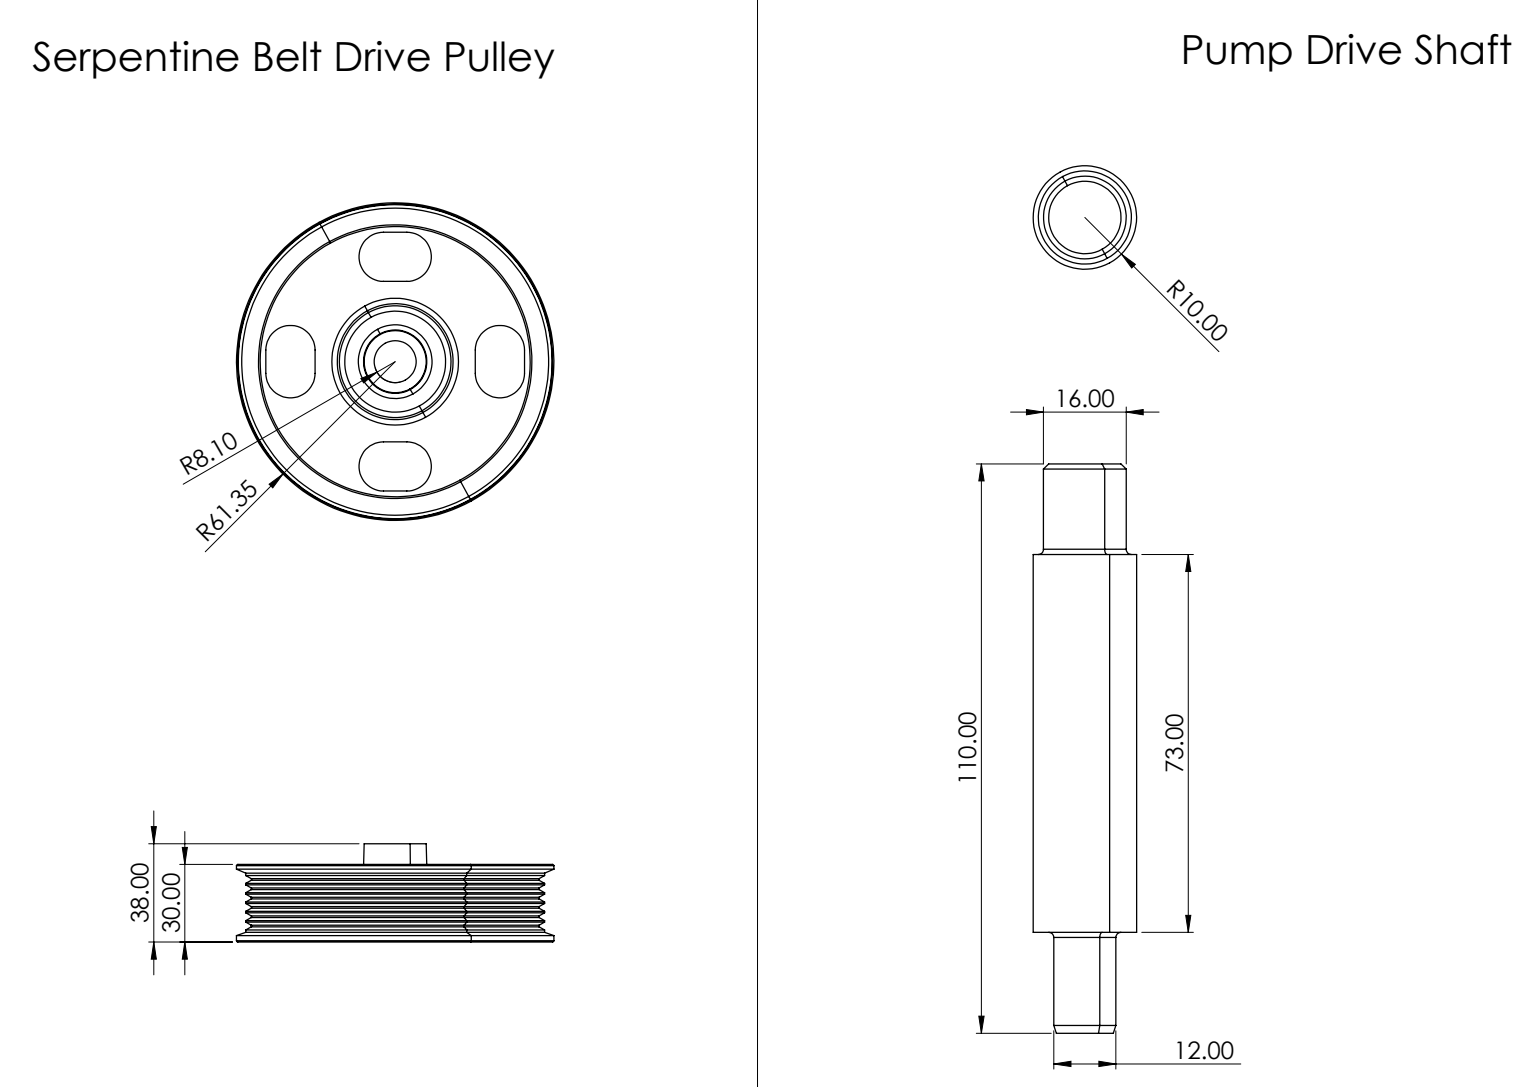
ISO-10303-21;
HEADER;
FILE_DESCRIPTION (('STEP AP214'),
    '1' );
FILE_NAME ('Pump Drive Shaft.step',
    '2026-10-09T13:19:41',
    ( '' ),
    ( '' ),
    'SwSTEP 2.0',
    'SolidWorks 2026',
    '' );
FILE_SCHEMA (( 'AUTOMOTIVE_DESIGN' ));
ENDSEC;

DATA;
#39=AXIS2_PLACEMENT_3D ( 'NONE', #26145, #6457, #10384 ) ;
#47=EDGE_CURVE ( 'NONE', #418, #1224, #23072, .T. ) ;
#183=CARTESIAN_POINT ( 'NONE',  ( 0.000000000000000000, 4.440892098500000496E-16, 0.000000000000000000 ) ) ;
#309=EDGE_LOOP ( 'NONE', ( #11613, #26788, #16517, #882 ) ) ;
#314=DIRECTION ( 'NONE',  ( 0.000000000000000000, -1.000000000000000000, 0.000000000000000000 ) ) ;
#372=DIRECTION ( 'NONE',  ( 0.000000000000000000, 1.000000000000000000, 0.000000000000000000 ) ) ;
#400=VERTEX_POINT ( 'NONE', #13649 ) ;
#418=VERTEX_POINT ( 'NONE', #2300 ) ;
#420=CARTESIAN_POINT ( 'NONE',  ( 0.000000000000000000, -90.50000000000000000, 0.000000000000000000 ) ) ;
#477=CYLINDRICAL_SURFACE ( 'NONE', #16417, 5.999999999999999112 ) ;
#489=LINE ( 'NONE', #22764, #1160 ) ;
#536=CONICAL_SURFACE ( 'NONE', #26096, 7.000000000000005329, 0.7853981633970000820 ) ;
#605=ADVANCED_FACE ( 'NONE', ( #18903 ), #27359, .T. ) ;
#882=ORIENTED_EDGE ( 'NONE', *, *, #11910, .F. ) ;
#893=CARTESIAN_POINT ( 'NONE',  ( -4.314829847440000421, -16.50000000000000000, -7.898243057010000179 ) ) ;
#942=VECTOR ( 'NONE', #24106, 999.9999999999998863 ) ;
#989=ORIENTED_EDGE ( 'NONE', *, *, #21743, .T. ) ;
#1012=CYLINDRICAL_SURFACE ( 'NONE', #26910, 9.999999999999996447 ) ;
#1058=DIRECTION ( 'NONE',  ( 0.000000000000000000, 1.000000000000000000, 0.000000000000000000 ) ) ;
#1160=VECTOR ( 'NONE', #22914, 1000.000000000000000 ) ;
#1187=VERTEX_POINT ( 'NONE', #12940 ) ;
#1224=VERTEX_POINT ( 'NONE', #14279 ) ;
#1275=DIRECTION ( 'NONE',  ( 1.000000000000000000, 0.000000000000000000, 0.000000000000000000 ) ) ;
#1309=PRODUCT ( 'Pump Drive Shaft', 'Pump Drive Shaft', '', ( #7289 ) ) ;
#1335=CARTESIAN_POINT ( 'NONE',  ( 0.000000000000000000, -90.50000000000000000, 0.000000000000000000 ) ) ;
#1353=DIRECTION ( 'NONE',  ( 0.4794255386042041156, 0.000000000000000000, 0.8775825618903722036 ) ) ;
#1356=LINE ( 'NONE', #11841, #17621 ) ;
#1363=ORIENTED_EDGE ( 'NONE', *, *, #7055, .F. ) ;
#1508=ORIENTED_EDGE ( 'NONE', *, *, #11910, .T. ) ;
#1532=ORIENTED_EDGE ( 'NONE', *, *, #17302, .F. ) ;
#1603=CONICAL_SURFACE ( 'NONE', #17400, 5.499999999999999112, 0.3217505543970000104 ) ;
#1714=FACE_OUTER_BOUND ( 'NONE', #309, .T. ) ;
#1771=DIRECTION ( 'NONE',  ( 0.000000000000000000, 1.000000000000000000, 0.000000000000000000 ) ) ;
#1915=DIRECTION ( 'NONE',  ( 0.000000000000000000, 1.000000000000000000, 0.000000000000000000 ) ) ;
#2006=SURFACE_STYLE_USAGE ( .BOTH. , #21957 ) ;
#2018=SHAPE_REPRESENTATION ( 'Pump Drive Shaft', ( #26433 ), #4100 ) ;
#2091=ADVANCED_FACE ( 'NONE', ( #11496 ), #477, .T. ) ;
#2175=CARTESIAN_POINT ( 'NONE',  ( 0.000000000000000000, -17.50000000000000000, 9.000000000000000000 ) ) ;
#2277=ADVANCED_FACE ( 'NONE', ( #17754 ), #24157, .F. ) ;
#2300=CARTESIAN_POINT ( 'NONE',  ( -2.636840462319999912, -110.0000000000000000, -4.826704090399999814 ) ) ;
#2315=ORIENTED_EDGE ( 'NONE', *, *, #7596, .T. ) ;
#2374=DIRECTION ( 'NONE',  ( 0.000000000000000000, 1.000000000000000000, 0.000000000000000000 ) ) ;
#2485=LINE ( 'NONE', #11341, #28396 ) ;
#2669=( NAMED_UNIT ( * ) PLANE_ANGLE_UNIT ( ) SI_UNIT ( $, .RADIAN. ) );
#2893=CONICAL_SURFACE ( 'NONE', #7090, 5.499999999999999112, 0.3217505543970000104 ) ;
#2930=CARTESIAN_POINT ( 'NONE',  ( -3.595691539529999758, -0.5000000000000000000, -6.581869214180000149 ) ) ;
#2950=DIRECTION ( 'NONE',  ( 0.000000000000000000, 1.000000000000000000, 0.000000000000000000 ) ) ;
#3005=AXIS2_PLACEMENT_3D ( 'NONE', #25732, #25170, #16694 ) ;
#3020=ORIENTED_EDGE ( 'NONE', *, *, #21743, .F. ) ;
#3033=EDGE_LOOP ( 'NONE', ( #27867, #12027, #6228, #27507 ) ) ;
#3034=AXIS2_PLACEMENT_3D ( 'NONE', #12319, #16700, #27659 ) ;
#3057=CARTESIAN_POINT ( 'NONE',  ( 0.000000000000000000, -90.50000000000000000, 0.000000000000000000 ) ) ;
#3314=AXIS2_PLACEMENT_3D ( 'NONE', #893, #16880, #19198 ) ;
#3446=CIRCLE ( 'NONE', #15027, 6.000000000000000000 ) ;
#3603=DIRECTION ( 'NONE',  ( 0.4794255386042040601, 0.000000000000000000, 0.8775825618903720926 ) ) ;
#3619=PRODUCT_DEFINITION_CONTEXT ( 'detailed design', #11839, 'design' ) ;
#3643=DIRECTION ( 'NONE',  ( 0.000000000000000000, 1.000000000000000000, 0.000000000000000000 ) ) ;
#3653=PRODUCT_DEFINITION_FORMATION_WITH_SPECIFIED_SOURCE ( 'ANY', '', #1309, .NOT_KNOWN. ) ;
#3670=ORIENTED_EDGE ( 'NONE', *, *, #26322, .F. ) ;
#3706=DIRECTION ( 'NONE',  ( 0.000000000000000000, 1.000000000000000000, 0.000000000000000000 ) ) ;
#3751=CARTESIAN_POINT ( 'NONE',  ( 0.000000000000000000, -110.0000000000000000, 0.000000000000000000 ) ) ;
#3889=DIRECTION ( 'NONE',  ( 1.000000000000000000, 0.000000000000000000, 0.000000000000000000 ) ) ;
#4040=ORIENTED_EDGE ( 'NONE', *, *, #20407, .T. ) ;
#4065=ADVANCED_FACE ( 'NONE', ( #10873, #19783 ), #17613, .T. ) ;
#4100=( GEOMETRIC_REPRESENTATION_CONTEXT ( 3 ) GLOBAL_UNCERTAINTY_ASSIGNED_CONTEXT ( ( #25217 ) ) GLOBAL_UNIT_ASSIGNED_CONTEXT ( ( #7186, #2669, #27289 ) ) REPRESENTATION_CONTEXT ( 'NONE', 'WORKASPACE' ) );
#4149=DIRECTION ( 'NONE',  ( 1.000000000000000000, 0.000000000000000000, 0.000000000000000000 ) ) ;
#4189=AXIS2_PLACEMENT_3D ( 'NONE', #19021, #12432, #23257 ) ;
#4211=DIRECTION ( 'NONE',  ( 0.000000000000000000, 1.000000000000000000, 0.000000000000000000 ) ) ;
#4213=TOROIDAL_SURFACE ( 'NONE', #5625, 9.000000000000000000, 1.000000000000000000 ) ;
#4271=VERTEX_POINT ( 'NONE', #17004 ) ;
#4384=DIRECTION ( 'NONE',  ( 0.000000000000000000, 1.000000000000000000, 0.000000000000000000 ) ) ;
#4492=DIRECTION ( 'NONE',  ( 0.4794255386042036715, 0.000000000000000000, 0.8775825618903724257 ) ) ;
#4610=ORIENTED_EDGE ( 'NONE', *, *, #24145, .F. ) ;
#4642=FACE_OUTER_BOUND ( 'NONE', #3033, .T. ) ;
#4769=VERTEX_POINT ( 'NONE', #9862 ) ;
#4778=ORIENTED_EDGE ( 'NONE', *, *, #20355, .F. ) ;
#4784=VERTEX_POINT ( 'NONE', #6974 ) ;
#4813=AXIS2_PLACEMENT_3D ( 'NONE', #183, #4384, #22460 ) ;
#4816=EDGE_LOOP ( 'NONE', ( #20575, #7039 ) ) ;
#4866=DIRECTION ( 'NONE',  ( 0.4794255386042041156, 0.000000000000000000, 0.8775825618903722036 ) ) ;
#5178=DIRECTION ( 'NONE',  ( 1.000000000000000000, 0.000000000000000000, 0.000000000000000000 ) ) ;
#5246=ORIENTED_EDGE ( 'NONE', *, *, #8164, .T. ) ;
#5297=FACE_OUTER_BOUND ( 'NONE', #22057, .T. ) ;
#5300=AXIS2_PLACEMENT_3D ( 'NONE', #17761, #26647, #4492 ) ;
#5306=ORIENTED_EDGE ( 'NONE', *, *, #15873, .T. ) ;
#5347=DIRECTION ( 'NONE',  ( 1.000000000000000000, 0.000000000000000000, 0.000000000000000000 ) ) ;
#5369=DIRECTION ( 'NONE',  ( 1.000000000000000000, 0.000000000000000000, 0.000000000000000000 ) ) ;
#5479=FACE_OUTER_BOUND ( 'NONE', #13459, .T. ) ;
#5542=DIRECTION ( 'NONE',  ( 0.000000000000000000, -1.000000000000000000, 0.000000000000000000 ) ) ;
#5562=DIRECTION ( 'NONE',  ( 0.000000000000000000, 0.000000000000000000, 1.000000000000000000 ) ) ;
#5625=AXIS2_PLACEMENT_3D ( 'NONE', #9053, #2374, #19834 ) ;
#5690=LINE ( 'NONE', #25390, #19752 ) ;
#5716=DIRECTION ( 'NONE',  ( 0.000000000000000000, -1.000000000000000000, 0.000000000000000000 ) ) ;
#5775=CONICAL_SURFACE ( 'NONE', #24864, 7.000000000000005329, 0.7853981633970000820 ) ;
#5779=ADVANCED_FACE ( 'NONE', ( #19274 ), #14250, .F. ) ;
#5873=APPLICATION_CONTEXT ( 'automotive_design' ) ;
#5923=CARTESIAN_POINT ( 'NONE',  ( 0.000000000000000000, -17.50000000000000000, 0.000000000000000000 ) ) ;
#6063=DIRECTION ( 'NONE',  ( 0.000000000000000000, 1.000000000000000000, 0.000000000000000000 ) ) ;
#6187=VERTEX_POINT ( 'NONE', #21283 ) ;
#6220=DIRECTION ( 'NONE',  ( 1.000000000000000000, 0.000000000000000000, 0.000000000000000000 ) ) ;
#6228=ORIENTED_EDGE ( 'NONE', *, *, #20978, .T. ) ;
#6355=( LENGTH_UNIT ( ) NAMED_UNIT ( * ) SI_UNIT ( .MILLI., .METRE. ) );
#6403=ORIENTED_EDGE ( 'NONE', *, *, #27600, .F. ) ;
#6415=EDGE_LOOP ( 'NONE', ( #22091, #8020, #14355, #23311 ) ) ;
#6422=AXIS2_PLACEMENT_3D ( 'NONE', #2175, #6539, #15399 ) ;
#6434=ORIENTED_EDGE ( 'NONE', *, *, #26155, .F. ) ;
#6457=DIRECTION ( 'NONE',  ( 0.000000000000000000, 1.000000000000000000, 0.000000000000000000 ) ) ;
#6485=DIRECTION ( 'NONE',  ( 0.000000000000000000, 1.000000000000000000, 0.000000000000000000 ) ) ;
#6516=VERTEX_POINT ( 'NONE', #18869 ) ;
#6536=DIRECTION ( 'NONE',  ( 0.000000000000000000, 1.000000000000000000, 0.000000000000000000 ) ) ;
#6539=DIRECTION ( 'NONE',  ( -0.000000000000000000, 1.000000000000000000, 0.000000000000000000 ) ) ;
#6576=VECTOR ( 'NONE', #27650, 999.9999999999998863 ) ;
#6581=DIRECTION ( 'NONE',  ( 1.000000000000000000, 0.000000000000000000, 0.000000000000000000 ) ) ;
#6816=DIRECTION ( 'NONE',  ( 0.000000000000000000, 1.000000000000000000, 0.000000000000000000 ) ) ;
#6896=EDGE_LOOP ( 'NONE', ( #23084, #27395, #25077, #1532 ) ) ;
#6906=ORIENTED_EDGE ( 'NONE', *, *, #6966, .T. ) ;
#6966=EDGE_CURVE ( 'NONE', #24664, #25480, #24285, .T. ) ;
#6974=CARTESIAN_POINT ( 'NONE',  ( -3.835404308829999831, -16.50000000000000000, -7.020660495120000455 ) ) ;
#7039=ORIENTED_EDGE ( 'NONE', *, *, #26322, .T. ) ;
#7044=AXIS2_PLACEMENT_3D ( 'NONE', #22912, #2950, #20725 ) ;
#7055=EDGE_CURVE ( 'NONE', #8407, #10083, #27854, .T. ) ;
#7090=AXIS2_PLACEMENT_3D ( 'NONE', #3751, #6063, #14942 ) ;
#7186=( LENGTH_UNIT ( ) NAMED_UNIT ( * ) SI_UNIT ( .MILLI., .METRE. ) );
#7192=COLOUR_RGB ( '', 0.08235294, 0.09019608, 0.10196078) ;
#7257=EDGE_CURVE ( 'NONE', #13019, #4784, #1356, .T. ) ;
#7289=PRODUCT_CONTEXT ( 'NONE', #5873, 'mechanical' ) ;
#7294=ADVANCED_FACE ( 'NONE', ( #21722 ), #14998, .T. ) ;
#7333=EDGE_LOOP ( 'NONE', ( #20871, #10302, #24906, #9615 ) ) ;
#7553=DIRECTION ( 'NONE',  ( 0.000000000000000000, 1.000000000000000000, 0.000000000000000000 ) ) ;
#7596=EDGE_CURVE ( 'NONE', #12424, #21733, #10605, .T. ) ;
#7643=TOROIDAL_SURFACE ( 'NONE', #5300, 7.000000000000000000, 1.000000000000000000 ) ;
#7677=AXIS2_PLACEMENT_3D ( 'NONE', #9584, #1915, #15275 ) ;
#7751=EDGE_CURVE ( 'NONE', #400, #1187, #20350, .T. ) ;
#7885=DIRECTION ( 'NONE',  ( 1.000000000000000000, 0.000000000000000000, 0.000000000000000000 ) ) ;
#7897=ORIENTED_EDGE ( 'NONE', *, *, #19984, .T. ) ;
#7923=CARTESIAN_POINT ( 'NONE',  ( 0.000000000000000000, -16.50000000000000000, 0.000000000000000000 ) ) ;
#7933=CIRCLE ( 'NONE', #39, 8.000000000000000000 ) ;
#8020=ORIENTED_EDGE ( 'NONE', *, *, #14353, .T. ) ;
#8064=CARTESIAN_POINT ( 'NONE',  ( 3.355978770230000130, 4.440892098500000496E-16, 6.143077933229999843 ) ) ;
#8112=ADVANCED_BREP_SHAPE_REPRESENTATION ( '', ( #25398, #26433 ), #4100 ) ;
#8120=SURFACE_STYLE_FILL_AREA ( #13046 ) ;
#8158=ADVANCED_FACE ( 'NONE', ( #14366, #5479 ), #24585, .F. ) ;
#8164=EDGE_CURVE ( 'NONE', #4271, #18220, #16246, .T. ) ;
#8253=DIRECTION ( 'NONE',  ( 0.000000000000000000, 1.000000000000000000, 0.000000000000000000 ) ) ;
#8355=DIRECTION ( 'NONE',  ( 0.000000000000000000, -1.000000000000000000, 0.000000000000000000 ) ) ;
#8363=VECTOR ( 'NONE', #8712, 1000.000000000000000 ) ;
#8387=( NAMED_UNIT ( * ) SI_UNIT ( $, .STERADIAN. ) SOLID_ANGLE_UNIT ( ) );
#8407=VERTEX_POINT ( 'NONE', #21362 ) ;
#8430=DIRECTION ( 'NONE',  ( 1.000000000000000000, 0.000000000000000000, 0.000000000000000000 ) ) ;
#8444=CIRCLE ( 'NONE', #22906, 9.000000000000000000 ) ;
#8447=EDGE_LOOP ( 'NONE', ( #9986, #1508, #23940, #6403 ) ) ;
#8512=ADVANCED_FACE ( 'NONE', ( #15794 ), #18140, .T. ) ;
#8549=DIRECTION ( 'NONE',  ( -0.000000000000000000, 1.000000000000000000, 0.000000000000000000 ) ) ;
#8712=DIRECTION ( 'NONE',  ( 0.000000000000000000, -1.000000000000000000, 0.000000000000000000 ) ) ;
#8840=CIRCLE ( 'NONE', #3314, 0.9999999999999997780 ) ;
#8976=DIRECTION ( 'NONE',  ( 0.000000000000000000, 1.000000000000000000, 0.000000000000000000 ) ) ;
#9053=CARTESIAN_POINT ( 'NONE',  ( 0.000000000000000000, -16.50000000000000000, 0.000000000000000000 ) ) ;
#9194=FACE_OUTER_BOUND ( 'NONE', #7333, .T. ) ;
#9414=ORIENTED_EDGE ( 'NONE', *, *, #7751, .T. ) ;
#9584=CARTESIAN_POINT ( 'NONE',  ( 0.000000000000000000, -1.000000000000000000, 0.000000000000000000 ) ) ;
#9608=CARTESIAN_POINT ( 'NONE',  ( -4.794255386040000566, -17.50000000000000000, -8.775825618900000791 ) ) ;
#9615=ORIENTED_EDGE ( 'NONE', *, *, #7596, .F. ) ;
#9756=DIRECTION ( 'NONE',  ( 0.4794255386042041156, 0.000000000000000000, 0.8775825618903722036 ) ) ;
#9802=CARTESIAN_POINT ( 'NONE',  ( 0.000000000000000000, 4.440892098500000496E-16, 0.000000000000000000 ) ) ;
#9862=CARTESIAN_POINT ( 'NONE',  ( 4.794255386040000566, -17.50000000000000000, 8.775825618900000791 ) ) ;
#9907=ADVANCED_FACE ( 'NONE', ( #5297 ), #18704, .T. ) ;
#9986=ORIENTED_EDGE ( 'NONE', *, *, #27633, .F. ) ;
#10009=ORIENTED_EDGE ( 'NONE', *, *, #26448, .F. ) ;
#10083=VERTEX_POINT ( 'NONE', #16025 ) ;
#10116=VECTOR ( 'NONE', #11793, 1000.000000000000114 ) ;
#10302=ORIENTED_EDGE ( 'NONE', *, *, #26155, .T. ) ;
#10384=DIRECTION ( 'NONE',  ( 1.000000000000000000, 0.000000000000000000, 0.000000000000000000 ) ) ;
#10444=CARTESIAN_POINT ( 'NONE',  ( 4.314829847440000421, -16.50000000000000000, 7.898243057010000179 ) ) ;
#10472=DIRECTION ( 'NONE',  ( -0.8775825618903722036, 0.000000000000000000, 0.4794255386042041156 ) ) ;
#10499=ADVANCED_FACE ( 'NONE', ( #9194 ), #4213, .F. ) ;
#10517=FACE_OUTER_BOUND ( 'NONE', #26931, .T. ) ;
#10546=DIRECTION ( 'NONE',  ( 0.000000000000000000, 1.000000000000000000, 0.000000000000000000 ) ) ;
#10605=CIRCLE ( 'NONE', #14387, 1.000000000000000444 ) ;
#10742=PRODUCT_DEFINITION ( 'UNKNOWN', '', #3653, #3619 ) ;
#10873=FACE_BOUND ( 'NONE', #23002, .T. ) ;
#11004=AXIS2_PLACEMENT_3D ( 'NONE', #28041, #3706, #12568 ) ;
#11007=CARTESIAN_POINT ( 'NONE',  ( 0.000000000000000000, -90.50000000000000000, 0.000000000000000000 ) ) ;
#11164=AXIS2_PLACEMENT_3D ( 'NONE', #420, #8976, #17883 ) ;
#11187=UNCERTAINTY_MEASURE_WITH_UNIT (LENGTH_MEASURE( 1.000000000000000082E-05 ), #6355, 'distance_accuracy_value', 'NONE');
#11341=CARTESIAN_POINT ( 'NONE',  ( 4.794255386040000566, -54.00000000000000000, 8.775825618900000791 ) ) ;
#11472=ORIENTED_EDGE ( 'NONE', *, *, #12195, .T. ) ;
#11496=FACE_OUTER_BOUND ( 'NONE', #17677, .T. ) ;
#11613=ORIENTED_EDGE ( 'NONE', *, *, #24788, .F. ) ;
#11780=EDGE_CURVE ( 'NONE', #12588, #4769, #13083, .T. ) ;
#11793=DIRECTION ( 'NONE',  ( -0.3390050494208429743, -0.7071067811866730279, -0.6205445805637129775 ) ) ;
#11815=CARTESIAN_POINT ( 'NONE',  ( 0.000000000000000000, 4.440892098500000496E-16, 0.000000000000000000 ) ) ;
#11827=ORIENTED_EDGE ( 'NONE', *, *, #15873, .F. ) ;
#11839=APPLICATION_CONTEXT ( 'automotive_design' ) ;
#11841=CARTESIAN_POINT ( 'NONE',  ( -3.835404308829999831, -8.750000000000000000, -7.020660495120000455 ) ) ;
#11886=EDGE_LOOP ( 'NONE', ( #15297, #14245, #989, #16793 ) ) ;
#11910=EDGE_CURVE ( 'NONE', #14582, #1224, #13309, .T. ) ;
#11912=DIRECTION ( 'NONE',  ( 0.000000000000000000, 1.000000000000000000, 0.000000000000000000 ) ) ;
#11982=AXIS2_PLACEMENT_3D ( 'NONE', #11007, #6536, #22267 ) ;
#12027=ORIENTED_EDGE ( 'NONE', *, *, #23379, .T. ) ;
#12039=VECTOR ( 'NONE', #5542, 1000.000000000000000 ) ;
#12099=ORIENTED_EDGE ( 'NONE', *, *, #24953, .F. ) ;
#12113=EDGE_LOOP ( 'NONE', ( #3670, #7897, #18361, #17927 ) ) ;
#12173=FACE_OUTER_BOUND ( 'NONE', #13167, .T. ) ;
#12195=EDGE_CURVE ( 'NONE', #25480, #14582, #14559, .T. ) ;
#12319=CARTESIAN_POINT ( 'NONE',  ( 0.000000000000000000, 0.000000000000000000, 0.000000000000000000 ) ) ;
#12369=DIRECTION ( 'NONE',  ( 1.000000000000000000, 0.000000000000000000, 0.000000000000000000 ) ) ;
#12424=VERTEX_POINT ( 'NONE', #22716 ) ;
#12432=DIRECTION ( 'NONE',  ( 0.000000000000000000, 1.000000000000000000, 0.000000000000000000 ) ) ;
#12568=DIRECTION ( 'NONE',  ( 1.000000000000000000, 0.000000000000000000, 0.000000000000000000 ) ) ;
#12576=EDGE_CURVE ( 'NONE', #4271, #13019, #19656, .T. ) ;
#12588=VERTEX_POINT ( 'NONE', #9608 ) ;
#12933=ADVANCED_FACE ( 'NONE', ( #25463 ), #1012, .T. ) ;
#12940=CARTESIAN_POINT ( 'NONE',  ( -3.355978770230000130, -90.50000000000000000, -6.143077933229999843 ) ) ;
#13008=EDGE_CURVE ( 'NONE', #1224, #418, #26416, .T. ) ;
#13019=VERTEX_POINT ( 'NONE', #15197 ) ;
#13038=CIRCLE ( 'NONE', #16796, 10.00000000000000000 ) ;
#13046=FILL_AREA_STYLE ('',( #24282 ) ) ;
#13083=CIRCLE ( 'NONE', #28002, 10.00000000000000000 ) ;
#13098=CIRCLE ( 'NONE', #17786, 9.000000000000000000 ) ;
#13167=EDGE_LOOP ( 'NONE', ( #10009, #16315, #6906, #19191 ) ) ;
#13207=MECHANICAL_DESIGN_GEOMETRIC_PRESENTATION_REPRESENTATION('',(#23473),#21152);
#13217=DIRECTION ( 'NONE',  ( -0.000000000000000000, 1.000000000000000000, 0.000000000000000000 ) ) ;
#13309=LINE ( 'NONE', #24401, #942 ) ;
#13383=AXIS2_PLACEMENT_3D ( 'NONE', #17274, #6485, #4149 ) ;
#13459=EDGE_LOOP ( 'NONE', ( #1363, #3020 ) ) ;
#13649=CARTESIAN_POINT ( 'NONE',  ( 3.355978770230000130, -90.50000000000000000, 6.143077933229999843 ) ) ;
#13772=ORIENTED_EDGE ( 'NONE', *, *, #7257, .F. ) ;
#13797=ORIENTED_EDGE ( 'NONE', *, *, #22100, .F. ) ;
#14030=CIRCLE ( 'NONE', #17215, 6.000000000000000000 ) ;
#14154=CARTESIAN_POINT ( 'NONE',  ( 2.876553231629999985, -108.5000000000000000, 5.265495371340000119 ) ) ;
#14184=DIRECTION ( 'NONE',  ( 0.000000000000000000, 1.000000000000000000, 0.000000000000000000 ) ) ;
#14245=ORIENTED_EDGE ( 'NONE', *, *, #27347, .T. ) ;
#14250=TOROIDAL_SURFACE ( 'NONE', #17963, 9.000000000000000000, 1.000000000000000000 ) ;
#14279=CARTESIAN_POINT ( 'NONE',  ( 2.636840462319999912, -110.0000000000000000, 4.826704090399999814 ) ) ;
#14299=DIRECTION ( 'NONE',  ( 0.000000000000000000, 1.000000000000000000, 0.000000000000000000 ) ) ;
#14353=EDGE_CURVE ( 'NONE', #24664, #6516, #24533, .T. ) ;
#14355=ORIENTED_EDGE ( 'NONE', *, *, #24788, .T. ) ;
#14366=FACE_BOUND ( 'NONE', #15613, .T. ) ;
#14383=DIRECTION ( 'NONE',  ( 0.4794255386042041711, 0.000000000000000000, 0.8775825618903722036 ) ) ;
#14387=AXIS2_PLACEMENT_3D ( 'NONE', #10444, #19222, #21688 ) ;
#14509=DIRECTION ( 'NONE',  ( 0.000000000000000000, 1.000000000000000000, 0.000000000000000000 ) ) ;
#14554=CIRCLE ( 'NONE', #18296, 0.9999999999999997780 ) ;
#14559=LINE ( 'NONE', #18673, #12039 ) ;
#14582=VERTEX_POINT ( 'NONE', #14154 ) ;
#14600=DIRECTION ( 'NONE',  ( 0.4794255386042036160, 0.000000000000000000, 0.8775825618903723147 ) ) ;
#14712=ORIENTED_EDGE ( 'NONE', *, *, #13008, .F. ) ;
#14846=DIRECTION ( 'NONE',  ( 0.8775825618903722036, 0.000000000000000000, -0.4794255386042041156 ) ) ;
#14942=DIRECTION ( 'NONE',  ( 0.4794255386042040601, 0.000000000000000000, 0.8775825618903720926 ) ) ;
#14998=CYLINDRICAL_SURFACE ( 'NONE', #24618, 5.999999999999999112 ) ;
#15027=AXIS2_PLACEMENT_3D ( 'NONE', #22028, #24497, #6581 ) ;
#15197=CARTESIAN_POINT ( 'NONE',  ( -3.835404308829999831, -1.000000000000000000, -7.020660495120000455 ) ) ;
#15255=AXIS2_PLACEMENT_3D ( 'NONE', #3057, #11912, #5369 ) ;
#15275=DIRECTION ( 'NONE',  ( 1.000000000000000000, 0.000000000000000000, 0.000000000000000000 ) ) ;
#15297=ORIENTED_EDGE ( 'NONE', *, *, #11780, .F. ) ;
#15362=CARTESIAN_POINT ( 'NONE',  ( -2.876553231629999985, -91.50000000000000000, -5.265495371340000119 ) ) ;
#15371=ORIENTED_EDGE ( 'NONE', *, *, #22553, .F. ) ;
#15399=DIRECTION ( 'NONE',  ( 1.000000000000000000, 0.000000000000000000, 0.000000000000000000 ) ) ;
#15511=TOROIDAL_SURFACE ( 'NONE', #3005, 7.000000000000000000, 1.000000000000000000 ) ;
#15551=ORIENTED_EDGE ( 'NONE', *, *, #16222, .F. ) ;
#15613=EDGE_LOOP ( 'NONE', ( #17320, #9414 ) ) ;
#15794=FACE_OUTER_BOUND ( 'NONE', #27542, .T. ) ;
#15827=ORIENTED_EDGE ( 'NONE', *, *, #24145, .T. ) ;
#15873=EDGE_CURVE ( 'NONE', #12424, #4784, #16629, .T. ) ;
#15893=DIRECTION ( 'NONE',  ( 0.000000000000000000, -1.000000000000000000, 0.000000000000000000 ) ) ;
#15904=AXIS2_PLACEMENT_3D ( 'NONE', #1335, #14299, #7885 ) ;
#16025=CARTESIAN_POINT ( 'NONE',  ( -4.794255386040000566, -90.50000000000000000, -8.775825618900000791 ) ) ;
#16222=EDGE_CURVE ( 'NONE', #25027, #13019, #16969, .T. ) ;
#16246=CIRCLE ( 'NONE', #22301, 7.000000000000000000 ) ;
#16315=ORIENTED_EDGE ( 'NONE', *, *, #18437, .T. ) ;
#16335=DIRECTION ( 'NONE',  ( 0.4794255386042036160, 0.000000000000000000, 0.8775825618903723147 ) ) ;
#16417=AXIS2_PLACEMENT_3D ( 'NONE', #18517, #1058, #9756 ) ;
#16466=ORIENTED_EDGE ( 'NONE', *, *, #7257, .T. ) ;
#16517=ORIENTED_EDGE ( 'NONE', *, *, #47, .T. ) ;
#16557=CARTESIAN_POINT ( 'NONE',  ( -2.756696846970000170, -109.2500000000000000, -5.046099730869999966 ) ) ;
#16629=CIRCLE ( 'NONE', #11004, 8.000000000000000000 ) ;
#16694=DIRECTION ( 'NONE',  ( 0.4794255386042036715, 0.000000000000000000, 0.8775825618903724257 ) ) ;
#16700=DIRECTION ( 'NONE',  ( 0.000000000000000000, 1.000000000000000000, 0.000000000000000000 ) ) ;
#16785=CARTESIAN_POINT ( 'NONE',  ( 0.000000000000000000, 0.000000000000000000, 0.000000000000000000 ) ) ;
#16793=ORIENTED_EDGE ( 'NONE', *, *, #19984, .F. ) ;
#16796=AXIS2_PLACEMENT_3D ( 'NONE', #19344, #8253, #6220 ) ;
#16807=DIRECTION ( 'NONE',  ( 0.000000000000000000, 1.000000000000000000, 0.000000000000000000 ) ) ;
#16828=ORIENTED_EDGE ( 'NONE', *, *, #27633, .T. ) ;
#16880=DIRECTION ( 'NONE',  ( 0.8775825618903722036, 0.000000000000000000, -0.4794255386042041156 ) ) ;
#16917=SHAPE_REPRESENTATION_RELATIONSHIP ( 'NONE' , 'NONE' ,  #2018, #8112 ) ;
#16969=CIRCLE ( 'NONE', #7677, 8.000000000000000000 ) ;
#17004=CARTESIAN_POINT ( 'NONE',  ( -3.355978770230000130, 4.440892098500000496E-16, -6.143077933229999843 ) ) ;
#17064=CARTESIAN_POINT ( 'NONE',  ( 0.000000000000000000, 0.000000000000000000, 0.000000000000000000 ) ) ;
#17215=AXIS2_PLACEMENT_3D ( 'NONE', #18896, #7553, #5347 ) ;
#17274=CARTESIAN_POINT ( 'NONE',  ( 0.000000000000000000, -110.0000000000000000, 0.000000000000000000 ) ) ;
#17302=EDGE_CURVE ( 'NONE', #18220, #25027, #5690, .T. ) ;
#17320=ORIENTED_EDGE ( 'NONE', *, *, #26448, .T. ) ;
#17362=CIRCLE ( 'NONE', #4813, 7.000000000000000000 ) ;
#17400=AXIS2_PLACEMENT_3D ( 'NONE', #27943, #10546, #3603 ) ;
#17451=DIRECTION ( 'NONE',  ( 1.000000000000000000, 0.000000000000000000, 0.000000000000000000 ) ) ;
#17613=PLANE ( 'NONE',  #6422 ) ;
#17621=VECTOR ( 'NONE', #21039, 1000.000000000000000 ) ;
#17677=EDGE_LOOP ( 'NONE', ( #20784, #11472, #16828, #27765 ) ) ;
#17754=FACE_OUTER_BOUND ( 'NONE', #21869, .T. ) ;
#17761=CARTESIAN_POINT ( 'NONE',  ( 0.000000000000000000, -91.50000000000000000, 0.000000000000000000 ) ) ;
#17786=AXIS2_PLACEMENT_3D ( 'NONE', #24028, #4211, #8430 ) ;
#17883=DIRECTION ( 'NONE',  ( 1.000000000000000000, 0.000000000000000000, 0.000000000000000000 ) ) ;
#17927=ORIENTED_EDGE ( 'NONE', *, *, #27347, .F. ) ;
#17963=AXIS2_PLACEMENT_3D ( 'NONE', #7923, #16807, #18997 ) ;
#17996=CARTESIAN_POINT ( 'NONE',  ( 0.000000000000000000, 0.000000000000000000, 0.000000000000000000 ) ) ;
#18038=CARTESIAN_POINT ( 'NONE',  ( 0.000000000000000000, -110.0000000000000000, 5.500000000000000000 ) ) ;
#18128=VECTOR ( 'NONE', #8355, 1000.000000000000000 ) ;
#18140=PLANE ( 'NONE',  #19498 ) ;
#18220=VERTEX_POINT ( 'NONE', #8064 ) ;
#18250=AXIS2_PLACEMENT_3D ( 'NONE', #18631, #27374, #20522 ) ;
#18296=AXIS2_PLACEMENT_3D ( 'NONE', #24041, #10472, #19665 ) ;
#18361=ORIENTED_EDGE ( 'NONE', *, *, #7055, .T. ) ;
#18437=EDGE_CURVE ( 'NONE', #1187, #24664, #19229, .T. ) ;
#18505=SHAPE_DEFINITION_REPRESENTATION ( #19666, #2018 ) ;
#18517=CARTESIAN_POINT ( 'NONE',  ( 0.000000000000000000, 0.000000000000000000, 0.000000000000000000 ) ) ;
#18631=CARTESIAN_POINT ( 'NONE',  ( 0.000000000000000000, -91.50000000000000000, 0.000000000000000000 ) ) ;
#18673=CARTESIAN_POINT ( 'NONE',  ( 2.876553231629999985, -100.0000000000000000, 5.265495371340000119 ) ) ;
#18681=CIRCLE ( 'NONE', #7044, 6.000000000000000000 ) ;
#18704=CYLINDRICAL_SURFACE ( 'NONE', #23752, 7.999999999999998224 ) ;
#18869=CARTESIAN_POINT ( 'NONE',  ( -2.876553231629999985, -108.5000000000000000, -5.265495371340000119 ) ) ;
#18896=CARTESIAN_POINT ( 'NONE',  ( 0.000000000000000000, -108.5000000000000000, 0.000000000000000000 ) ) ;
#18903=FACE_OUTER_BOUND ( 'NONE', #12113, .T. ) ;
#18957=CARTESIAN_POINT ( 'NONE',  ( 4.314829847440000421, -17.50000000000000000, 7.898243057010000179 ) ) ;
#18997=DIRECTION ( 'NONE',  ( 0.4794255386042041156, 0.000000000000000000, 0.8775825618903722036 ) ) ;
#19021=CARTESIAN_POINT ( 'NONE',  ( 0.000000000000000000, -1.000000000000000000, 0.000000000000000000 ) ) ;
#19177=DIRECTION ( 'NONE',  ( 0.000000000000000000, 1.000000000000000000, 0.000000000000000000 ) ) ;
#19191=ORIENTED_EDGE ( 'NONE', *, *, #23379, .F. ) ;
#19198=DIRECTION ( 'NONE',  ( 0.4794255386042042266, 0.000000000000000000, 0.8775825618903720926 ) ) ;
#19222=DIRECTION ( 'NONE',  ( -0.8775825618903722036, 0.000000000000000000, 0.4794255386042041156 ) ) ;
#19229=CIRCLE ( 'NONE', #26195, 0.9999999999999997780 ) ;
#19274=FACE_OUTER_BOUND ( 'NONE', #24449, .T. ) ;
#19344=CARTESIAN_POINT ( 'NONE',  ( 0.000000000000000000, -17.50000000000000000, 0.000000000000000000 ) ) ;
#19378=ADVANCED_FACE ( 'NONE', ( #28351 ), #1603, .T. ) ;
#19464=ORIENTED_EDGE ( 'NONE', *, *, #24953, .T. ) ;
#19467=( NAMED_UNIT ( * ) PLANE_ANGLE_UNIT ( ) SI_UNIT ( $, .RADIAN. ) );
#19498=AXIS2_PLACEMENT_3D ( 'NONE', #17996, #22525, #5178 ) ;
#19656=LINE ( 'NONE', #2930, #10116 ) ;
#19665=DIRECTION ( 'NONE',  ( 0.4794255386042042266, 0.000000000000000000, 0.8775825618903720926 ) ) ;
#19666=PRODUCT_DEFINITION_SHAPE ( 'NONE', 'NONE',  #10742 ) ;
#19752=VECTOR ( 'NONE', #21420, 1000.000000000000114 ) ;
#19783=FACE_OUTER_BOUND ( 'NONE', #4816, .T. ) ;
#19785=CLOSED_SHELL ( 'NONE', ( #2277, #19378, #22113, #2091, #7294, #24582, #25580, #8158, #605, #12933, #4065, #10499, #5779, #9907, #20583, #24984, #8512, #20706 ) ) ;
#19834=DIRECTION ( 'NONE',  ( 0.4794255386042041156, 0.000000000000000000, 0.8775825618903722036 ) ) ;
#19984=EDGE_CURVE ( 'NONE', #4769, #8407, #2485, .T. ) ;
#20350=CIRCLE ( 'NONE', #11982, 7.000000000000000000 ) ;
#20355=EDGE_CURVE ( 'NONE', #13019, #25027, #26537, .T. ) ;
#20407=EDGE_CURVE ( 'NONE', #4784, #12424, #7933, .T. ) ;
#20419=CARTESIAN_POINT ( 'NONE',  ( 3.835404308829999831, -1.000000000000000000, 7.020660495120000455 ) ) ;
#20500=CIRCLE ( 'NONE', #11164, 7.000000000000000000 ) ;
#20522=DIRECTION ( 'NONE',  ( 1.000000000000000000, 0.000000000000000000, 0.000000000000000000 ) ) ;
#20562=CIRCLE ( 'NONE', #15904, 10.00000000000000000 ) ;
#20575=ORIENTED_EDGE ( 'NONE', *, *, #11780, .T. ) ;
#20583=ADVANCED_FACE ( 'NONE', ( #10517 ), #22794, .T. ) ;
#20706=ADVANCED_FACE ( 'NONE', ( #28013 ), #536, .T. ) ;
#20725=DIRECTION ( 'NONE',  ( 1.000000000000000000, 0.000000000000000000, 0.000000000000000000 ) ) ;
#20784=ORIENTED_EDGE ( 'NONE', *, *, #20978, .F. ) ;
#20871=ORIENTED_EDGE ( 'NONE', *, *, #20407, .F. ) ;
#20978=EDGE_CURVE ( 'NONE', #25480, #24664, #18681, .T. ) ;
#21039=DIRECTION ( 'NONE',  ( 0.000000000000000000, -1.000000000000000000, 0.000000000000000000 ) ) ;
#21086=LINE ( 'NONE', #16557, #6576 ) ;
#21152=( GEOMETRIC_REPRESENTATION_CONTEXT ( 3 ) GLOBAL_UNCERTAINTY_ASSIGNED_CONTEXT ( ( #11187 ) ) GLOBAL_UNIT_ASSIGNED_CONTEXT ( ( #6355, #19467, #8387 ) ) REPRESENTATION_CONTEXT ( 'NONE', 'WORKASPACE' ) );
#21223=CARTESIAN_POINT ( 'NONE',  ( 0.000000000000000000, -17.50000000000000000, 0.000000000000000000 ) ) ;
#21283=CARTESIAN_POINT ( 'NONE',  ( -4.314829847440000421, -17.50000000000000000, -7.898243057010000179 ) ) ;
#21362=CARTESIAN_POINT ( 'NONE',  ( 4.794255386040000566, -90.50000000000000000, 8.775825618900000791 ) ) ;
#21363=CARTESIAN_POINT ( 'NONE',  ( 0.000000000000000000, 0.000000000000000000, 0.000000000000000000 ) ) ;
#21402=ORIENTED_EDGE ( 'NONE', *, *, #12576, .F. ) ;
#21420=DIRECTION ( 'NONE',  ( 0.3390050494208429743, -0.7071067811866730279, 0.6205445805637129775 ) ) ;
#21566=CARTESIAN_POINT ( 'NONE',  ( -3.355978770230000130, -91.50000000000000000, -6.143077933229999843 ) ) ;
#21584=DIRECTION ( 'NONE',  ( 0.4794255386042041156, 0.000000000000000000, 0.8775825618903722036 ) ) ;
#21688=DIRECTION ( 'NONE',  ( 0.4794255386042038936, 0.000000000000000000, 0.8775825618903723147 ) ) ;
#21722=FACE_OUTER_BOUND ( 'NONE', #6415, .T. ) ;
#21733=VERTEX_POINT ( 'NONE', #18957 ) ;
#21743=EDGE_CURVE ( 'NONE', #10083, #8407, #20562, .T. ) ;
#21804=PRESENTATION_STYLE_ASSIGNMENT (( #2006 ) ) ;
#21869=EDGE_LOOP ( 'NONE', ( #14712, #25672 ) ) ;
#21957=SURFACE_SIDE_STYLE ('',( #8120 ) ) ;
#22028=CARTESIAN_POINT ( 'NONE',  ( 0.000000000000000000, -108.5000000000000000, 0.000000000000000000 ) ) ;
#22057=EDGE_LOOP ( 'NONE', ( #4778, #16466, #4040, #12099 ) ) ;
#22069=CARTESIAN_POINT ( 'NONE',  ( -2.876553231629999985, -100.0000000000000000, -5.265495371340000119 ) ) ;
#22091=ORIENTED_EDGE ( 'NONE', *, *, #6966, .F. ) ;
#22100=EDGE_CURVE ( 'NONE', #6187, #21733, #8444, .T. ) ;
#22113=ADVANCED_FACE ( 'NONE', ( #1714 ), #2893, .T. ) ;
#22125=DIRECTION ( 'NONE',  ( 1.000000000000000000, 0.000000000000000000, 0.000000000000000000 ) ) ;
#22252=DIRECTION ( 'NONE',  ( 1.000000000000000000, 0.000000000000000000, 0.000000000000000000 ) ) ;
#22267=DIRECTION ( 'NONE',  ( 1.000000000000000000, 0.000000000000000000, 0.000000000000000000 ) ) ;
#22301=AXIS2_PLACEMENT_3D ( 'NONE', #26335, #6816, #22252 ) ;
#22460=DIRECTION ( 'NONE',  ( 1.000000000000000000, 0.000000000000000000, 0.000000000000000000 ) ) ;
#22525=DIRECTION ( 'NONE',  ( -0.000000000000000000, 1.000000000000000000, 0.000000000000000000 ) ) ;
#22553=EDGE_CURVE ( 'NONE', #21733, #6187, #13098, .T. ) ;
#22605=AXIS2_PLACEMENT_3D ( 'NONE', #26067, #3643, #12369 ) ;
#22617=FACE_OUTER_BOUND ( 'NONE', #6896, .T. ) ;
#22716=CARTESIAN_POINT ( 'NONE',  ( 3.835404308829999831, -16.50000000000000000, 7.020660495120000455 ) ) ;
#22764=CARTESIAN_POINT ( 'NONE',  ( 3.835404308829999831, -8.750000000000000000, 7.020660495120000455 ) ) ;
#22794=CYLINDRICAL_SURFACE ( 'NONE', #27033, 7.999999999999998224 ) ;
#22906=AXIS2_PLACEMENT_3D ( 'NONE', #5923, #26330, #3889 ) ;
#22912=CARTESIAN_POINT ( 'NONE',  ( 0.000000000000000000, -91.50000000000000000, 0.000000000000000000 ) ) ;
#22914=DIRECTION ( 'NONE',  ( 0.000000000000000000, -1.000000000000000000, 0.000000000000000000 ) ) ;
#23002=EDGE_LOOP ( 'NONE', ( #15371, #13797 ) ) ;
#23072=CIRCLE ( 'NONE', #22605, 5.500000000000000000 ) ;
#23084=ORIENTED_EDGE ( 'NONE', *, *, #8164, .F. ) ;
#23148=EDGE_LOOP ( 'NONE', ( #4610, #23727, #27113, #21402 ) ) ;
#23257=DIRECTION ( 'NONE',  ( 1.000000000000000000, 0.000000000000000000, 0.000000000000000000 ) ) ;
#23311=ORIENTED_EDGE ( 'NONE', *, *, #12195, .F. ) ;
#23379=EDGE_CURVE ( 'NONE', #400, #25480, #14554, .T. ) ;
#23473=STYLED_ITEM ( 'NONE', ( #21804 ), #25398 ) ;
#23727=ORIENTED_EDGE ( 'NONE', *, *, #17302, .T. ) ;
#23752=AXIS2_PLACEMENT_3D ( 'NONE', #16785, #14184, #1353 ) ;
#23940=ORIENTED_EDGE ( 'NONE', *, *, #13008, .T. ) ;
#24028=CARTESIAN_POINT ( 'NONE',  ( 0.000000000000000000, -17.50000000000000000, 0.000000000000000000 ) ) ;
#24041=CARTESIAN_POINT ( 'NONE',  ( 3.355978770230000130, -91.50000000000000000, 6.143077933229999843 ) ) ;
#24106=DIRECTION ( 'NONE',  ( -0.1516076670439319707, -0.9486832980505756074, -0.2775159730418759185 ) ) ;
#24145=EDGE_CURVE ( 'NONE', #18220, #4271, #17362, .T. ) ;
#24157=PLANE ( 'NONE',  #28498 ) ;
#24282=FILL_AREA_STYLE_COLOUR ( '', #7192 ) ;
#24285=CIRCLE ( 'NONE', #18250, 6.000000000000000000 ) ;
#24401=CARTESIAN_POINT ( 'NONE',  ( 2.756696846970000170, -109.2500000000000000, 5.046099730869999966 ) ) ;
#24449=EDGE_LOOP ( 'NONE', ( #11827, #2315, #27162, #6434 ) ) ;
#24475=LINE ( 'NONE', #28678, #8363 ) ;
#24497=DIRECTION ( 'NONE',  ( 0.000000000000000000, 1.000000000000000000, 0.000000000000000000 ) ) ;
#24533=LINE ( 'NONE', #22069, #18128 ) ;
#24582=ADVANCED_FACE ( 'NONE', ( #4642 ), #7643, .F. ) ;
#24585=PLANE ( 'NONE',  #28790 ) ;
#24618=AXIS2_PLACEMENT_3D ( 'NONE', #17064, #1771, #21584 ) ;
#24664=VERTEX_POINT ( 'NONE', #15362 ) ;
#24788=EDGE_CURVE ( 'NONE', #6516, #14582, #3446, .T. ) ;
#24864=AXIS2_PLACEMENT_3D ( 'NONE', #11815, #15893, #16335 ) ;
#24906=ORIENTED_EDGE ( 'NONE', *, *, #22100, .T. ) ;
#24953=EDGE_CURVE ( 'NONE', #25027, #12424, #489, .T. ) ;
#24972=CARTESIAN_POINT ( 'NONE',  ( 0.000000000000000000, 0.000000000000000000, 0.000000000000000000 ) ) ;
#24984=ADVANCED_FACE ( 'NONE', ( #22617 ), #5775, .T. ) ;
#25015=CARTESIAN_POINT ( 'NONE',  ( 2.876553231629999985, -91.50000000000000000, 5.265495371340000119 ) ) ;
#25027=VERTEX_POINT ( 'NONE', #20419 ) ;
#25077=ORIENTED_EDGE ( 'NONE', *, *, #20355, .T. ) ;
#25170=DIRECTION ( 'NONE',  ( 0.000000000000000000, 1.000000000000000000, 0.000000000000000000 ) ) ;
#25217=UNCERTAINTY_MEASURE_WITH_UNIT (LENGTH_MEASURE( 1.000000000000000082E-05 ), #7186, 'distance_accuracy_value', 'NONE');
#25255=DIRECTION ( 'NONE',  ( 1.000000000000000000, 0.000000000000000000, 0.000000000000000000 ) ) ;
#25390=CARTESIAN_POINT ( 'NONE',  ( 3.595691539529999758, -0.5000000000000000000, 6.581869214180000149 ) ) ;
#25398=MANIFOLD_SOLID_BREP ( 'Rotational Bodies', #19785 ) ;
#25463=FACE_OUTER_BOUND ( 'NONE', #11886, .T. ) ;
#25480=VERTEX_POINT ( 'NONE', #25015 ) ;
#25580=ADVANCED_FACE ( 'NONE', ( #12173 ), #15511, .F. ) ;
#25672=ORIENTED_EDGE ( 'NONE', *, *, #47, .F. ) ;
#25732=CARTESIAN_POINT ( 'NONE',  ( 0.000000000000000000, -91.50000000000000000, 0.000000000000000000 ) ) ;
#25939=DIRECTION ( 'NONE',  ( 0.4794255386042042266, 0.000000000000000000, 0.8775825618903720926 ) ) ;
#26067=CARTESIAN_POINT ( 'NONE',  ( 0.000000000000000000, -110.0000000000000000, 0.000000000000000000 ) ) ;
#26096=AXIS2_PLACEMENT_3D ( 'NONE', #9802, #5716, #14600 ) ;
#26145=CARTESIAN_POINT ( 'NONE',  ( 0.000000000000000000, -16.50000000000000000, 0.000000000000000000 ) ) ;
#26155=EDGE_CURVE ( 'NONE', #4784, #6187, #8840, .T. ) ;
#26195=AXIS2_PLACEMENT_3D ( 'NONE', #21566, #14846, #25939 ) ;
#26322=EDGE_CURVE ( 'NONE', #4769, #12588, #13038, .T. ) ;
#26330=DIRECTION ( 'NONE',  ( 0.000000000000000000, 1.000000000000000000, 0.000000000000000000 ) ) ;
#26335=CARTESIAN_POINT ( 'NONE',  ( 0.000000000000000000, 0.000000000000000000, 0.000000000000000000 ) ) ;
#26416=CIRCLE ( 'NONE', #13383, 5.500000000000000000 ) ;
#26433=AXIS2_PLACEMENT_3D ( 'NONE', #27589, #5562, #25255 ) ;
#26448=EDGE_CURVE ( 'NONE', #1187, #400, #20500, .T. ) ;
#26537=CIRCLE ( 'NONE', #4189, 8.000000000000000000 ) ;
#26628=CARTESIAN_POINT ( 'NONE',  ( 0.000000000000000000, -90.50000000000000000, 10.00000000000000000 ) ) ;
#26647=DIRECTION ( 'NONE',  ( 0.000000000000000000, 1.000000000000000000, 0.000000000000000000 ) ) ;
#26788=ORIENTED_EDGE ( 'NONE', *, *, #27600, .T. ) ;
#26910=AXIS2_PLACEMENT_3D ( 'NONE', #21363, #19177, #14383 ) ;
#26931=EDGE_LOOP ( 'NONE', ( #15551, #19464, #5306, #13772 ) ) ;
#27033=AXIS2_PLACEMENT_3D ( 'NONE', #24972, #372, #4866 ) ;
#27113=ORIENTED_EDGE ( 'NONE', *, *, #16222, .T. ) ;
#27162=ORIENTED_EDGE ( 'NONE', *, *, #22553, .T. ) ;
#27289=( NAMED_UNIT ( * ) SI_UNIT ( $, .STERADIAN. ) SOLID_ANGLE_UNIT ( ) );
#27347=EDGE_CURVE ( 'NONE', #12588, #10083, #24475, .T. ) ;
#27359=CYLINDRICAL_SURFACE ( 'NONE', #3034, 9.999999999999996447 ) ;
#27374=DIRECTION ( 'NONE',  ( 0.000000000000000000, 1.000000000000000000, 0.000000000000000000 ) ) ;
#27395=ORIENTED_EDGE ( 'NONE', *, *, #12576, .T. ) ;
#27507=ORIENTED_EDGE ( 'NONE', *, *, #18437, .F. ) ;
#27542=EDGE_LOOP ( 'NONE', ( #15827, #5246 ) ) ;
#27589=CARTESIAN_POINT ( 'NONE',  ( 0.000000000000000000, 0.000000000000000000, 0.000000000000000000 ) ) ;
#27600=EDGE_CURVE ( 'NONE', #6516, #418, #21086, .T. ) ;
#27633=EDGE_CURVE ( 'NONE', #14582, #6516, #14030, .T. ) ;
#27650=DIRECTION ( 'NONE',  ( 0.1516076670439319707, -0.9486832980505756074, 0.2775159730418759185 ) ) ;
#27659=DIRECTION ( 'NONE',  ( 0.4794255386042041711, 0.000000000000000000, 0.8775825618903722036 ) ) ;
#27765=ORIENTED_EDGE ( 'NONE', *, *, #14353, .F. ) ;
#27854=CIRCLE ( 'NONE', #15255, 10.00000000000000000 ) ;
#27867=ORIENTED_EDGE ( 'NONE', *, *, #7751, .F. ) ;
#27943=CARTESIAN_POINT ( 'NONE',  ( 0.000000000000000000, -110.0000000000000000, 0.000000000000000000 ) ) ;
#28002=AXIS2_PLACEMENT_3D ( 'NONE', #21223, #14509, #1275 ) ;
#28013=FACE_OUTER_BOUND ( 'NONE', #23148, .T. ) ;
#28041=CARTESIAN_POINT ( 'NONE',  ( 0.000000000000000000, -16.50000000000000000, 0.000000000000000000 ) ) ;
#28351=FACE_OUTER_BOUND ( 'NONE', #8447, .T. ) ;
#28396=VECTOR ( 'NONE', #314, 1000.000000000000000 ) ;
#28498=AXIS2_PLACEMENT_3D ( 'NONE', #18038, #13217, #22125 ) ;
#28678=CARTESIAN_POINT ( 'NONE',  ( -4.794255386040000566, -54.00000000000000000, -8.775825618900000791 ) ) ;
#28790=AXIS2_PLACEMENT_3D ( 'NONE', #26628, #8549, #17451 ) ;
ENDSEC;
END-ISO-10303-21;
